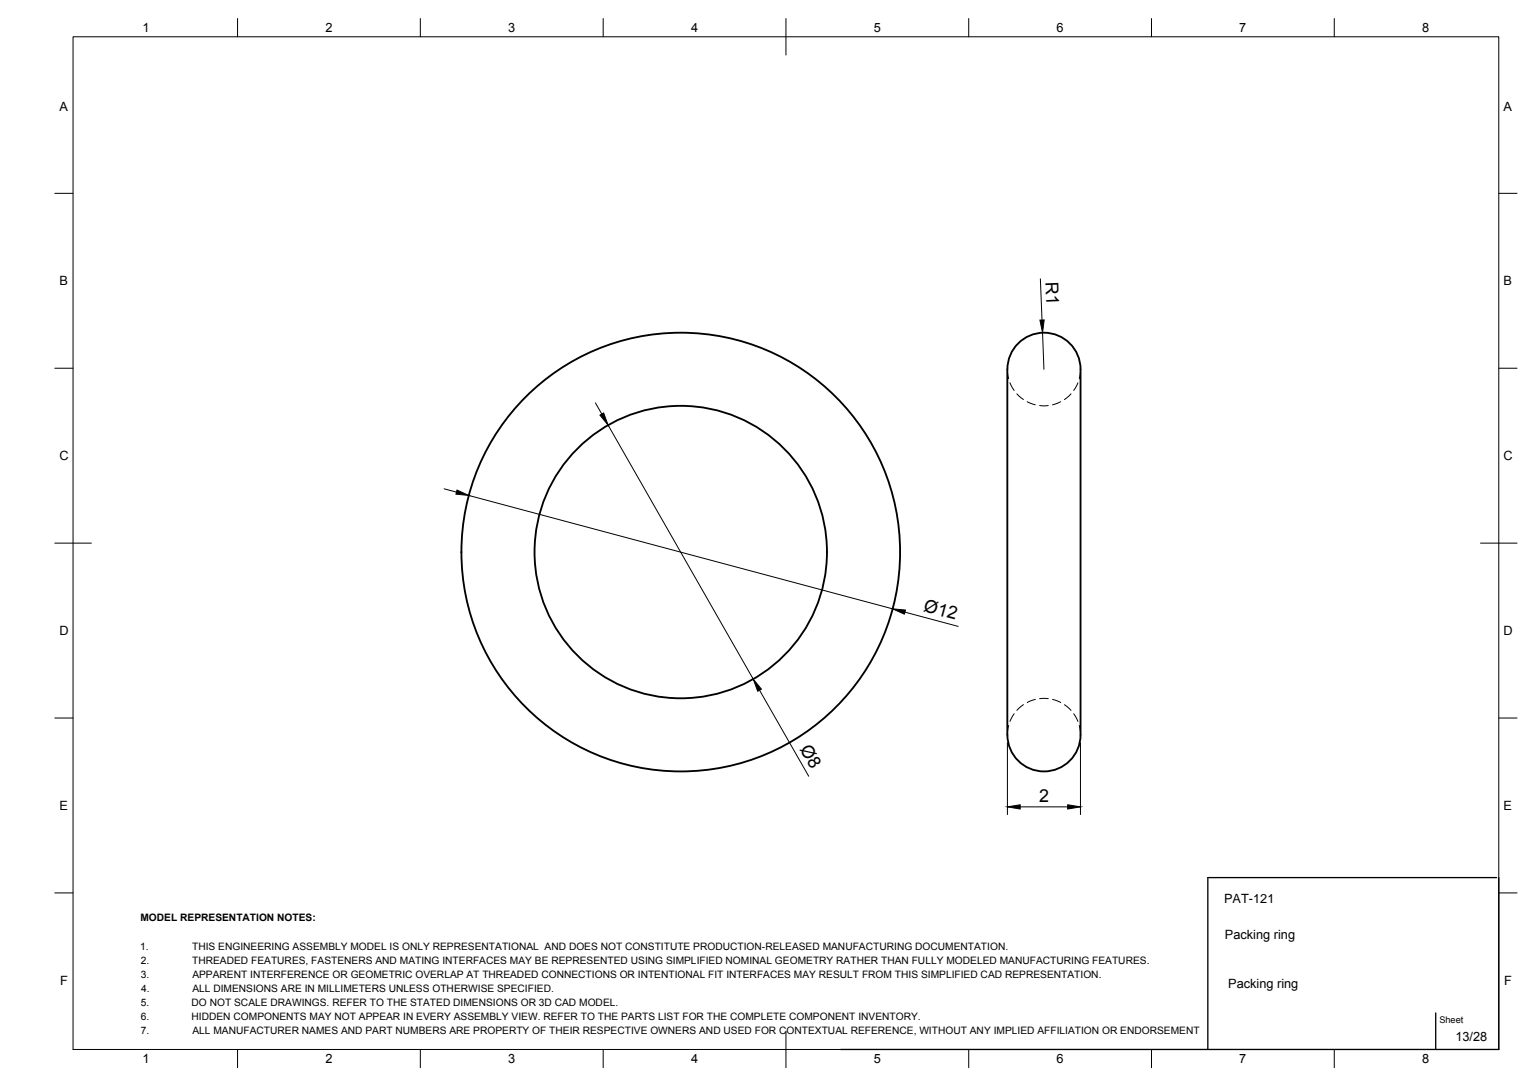
ISO-10303-21;
HEADER;
/* Generated by software containing ST-Developer
 * from STEP Tools, Inc. (www.steptools.com) 
 */

FILE_DESCRIPTION(
/* description */ ('Wall-mounted air drop station'),
/* implementation_level */ '2;1');

FILE_NAME(
/* name */ 'Packing ring.step',
/* time_stamp */ '2026-10-28T22:16:19-07:00',
/* author */ (''),
/* organization */ (''),
/* preprocessor_version */ 'ST-DEVELOPER v20.2',
/* originating_system */ 'Autodesk Translation Framework v15.17.0.0',
/* authorisation */ '');

FILE_SCHEMA (('AUTOMOTIVE_DESIGN { 1 0 10303 214 3 1 1 }'));
ENDSEC;

DATA;
#10=MECHANICAL_DESIGN_GEOMETRIC_PRESENTATION_REPRESENTATION('',(#353),#10517);
#257=TOROIDAL_SURFACE('',#6508,0.5,0.1);
#295=SHAPE_REPRESENTATION_RELATIONSHIP('SRR','None',#10652,#324);
#324=ADVANCED_BREP_SHAPE_REPRESENTATION('',(#382),#10496);
#353=STYLED_ITEM('',(#10867),#382);
#382=MANIFOLD_SOLID_BREP('Body1',#5892);
#902=FACE_OUTER_BOUND('',#1332,.T.);
#1332=EDGE_LOOP('',(#4609,#4610,#4611,#4612));
#2634=CIRCLE('',#6509,0.1);
#2635=CIRCLE('',#6510,0.4);
#2977=VERTEX_POINT('',#9456);
#3562=EDGE_CURVE('',#2977,#2977,#2634,.T.);
#3563=EDGE_CURVE('',#2977,#2977,#2635,.T.);
#4609=ORIENTED_EDGE('',*,*,#3562,.F.);
#4610=ORIENTED_EDGE('',*,*,#3563,.T.);
#4611=ORIENTED_EDGE('',*,*,#3562,.T.);
#4612=ORIENTED_EDGE('',*,*,#3563,.F.);
#5675=ADVANCED_FACE('',(#902),#257,.T.);
#5892=CLOSED_SHELL('',(#5675));
#6507=AXIS2_PLACEMENT_3D('',#9454,#7672,#7673);
#6508=AXIS2_PLACEMENT_3D('',#9455,#7674,#7675);
#6509=AXIS2_PLACEMENT_3D('',#9457,#7676,#7677);
#6510=AXIS2_PLACEMENT_3D('',#9458,#7678,#7679);
#7672=DIRECTION('axis',(0.,0.,1.));
#7673=DIRECTION('refdir',(1.,0.,0.));
#7674=DIRECTION('center_axis',(0.,0.,1.));
#7675=DIRECTION('ref_axis',(1.,0.,0.));
#7676=DIRECTION('center_axis',(1.22464679914735E-16,-1.,0.));
#7677=DIRECTION('ref_axis',(-1.,-1.22464679914735E-16,0.));
#7678=DIRECTION('center_axis',(0.,0.,-1.));
#7679=DIRECTION('ref_axis',(1.,0.,0.));
#9454=CARTESIAN_POINT('',(0.,0.,0.));
#9455=CARTESIAN_POINT('Origin',(0.,0.,8.1));
#9456=CARTESIAN_POINT('',(-0.4,-4.89858719658941E-17,8.1));
#9457=CARTESIAN_POINT('Origin',(-0.5,-6.12323399573677E-17,8.1));
#9458=CARTESIAN_POINT('Origin',(0.,0.,8.1));
#10463=UNCERTAINTY_MEASURE_WITH_UNIT(LENGTH_MEASURE(0.001),#10518,
'DISTANCE_ACCURACY_VALUE',
'Maximum model space distance between geometric entities at asserted c
onnectivities');
#10484=UNCERTAINTY_MEASURE_WITH_UNIT(LENGTH_MEASURE(0.001),#10518,
'DISTANCE_ACCURACY_VALUE',
'Maximum model space distance between geometric entities at asserted c
onnectivities');
#10496=(
GEOMETRIC_REPRESENTATION_CONTEXT(3)
GLOBAL_UNCERTAINTY_ASSIGNED_CONTEXT((#10463))
GLOBAL_UNIT_ASSIGNED_CONTEXT((#10518,#10520,#10521))
REPRESENTATION_CONTEXT('','3D')
);
#10517=(
GEOMETRIC_REPRESENTATION_CONTEXT(3)
GLOBAL_UNCERTAINTY_ASSIGNED_CONTEXT((#10484))
GLOBAL_UNIT_ASSIGNED_CONTEXT((#10518,#10520,#10521))
REPRESENTATION_CONTEXT('','3D')
);
#10518=(
LENGTH_UNIT()
NAMED_UNIT(*)
SI_UNIT(.CENTI.,.METRE.)
);
#10520=(
NAMED_UNIT(*)
PLANE_ANGLE_UNIT()
SI_UNIT($,.RADIAN.)
);
#10521=(
NAMED_UNIT(*)
SI_UNIT($,.STERADIAN.)
SOLID_ANGLE_UNIT()
);
#10533=SHAPE_DEFINITION_REPRESENTATION(#10565,#10652);
#10565=PRODUCT_DEFINITION_SHAPE('',$,#10685);
#10652=SHAPE_REPRESENTATION('',(#6507),#10496);
#10673=PRODUCT_DEFINITION_CONTEXT('part definition',#10771,'design');
#10685=PRODUCT_DEFINITION('Packing ring','Packing ring',#10717,#10673);
#10717=PRODUCT_DEFINITION_FORMATION('',$,#10784);
#10771=APPLICATION_CONTEXT(
'Core Data for Automotive Mechanical Design Process');
#10772=PRODUCT_CONTEXT('part definition',#10771,'mechanical');
#10784=PRODUCT('Packing ring','Packing ring','Packing ring',(#10772));
#10861=COLOUR_RGB('Sky Blue',0.24,0.69,0.87);
#10862=FILL_AREA_STYLE_COLOUR('',#10861);
#10863=FILL_AREA_STYLE('',(#10862));
#10864=SURFACE_STYLE_FILL_AREA(#10863);
#10865=SURFACE_SIDE_STYLE('',(#10864));
#10866=SURFACE_STYLE_USAGE(.BOTH.,#10865);
#10867=PRESENTATION_STYLE_ASSIGNMENT((#10866));
ENDSEC;
END-ISO-10303-21;
